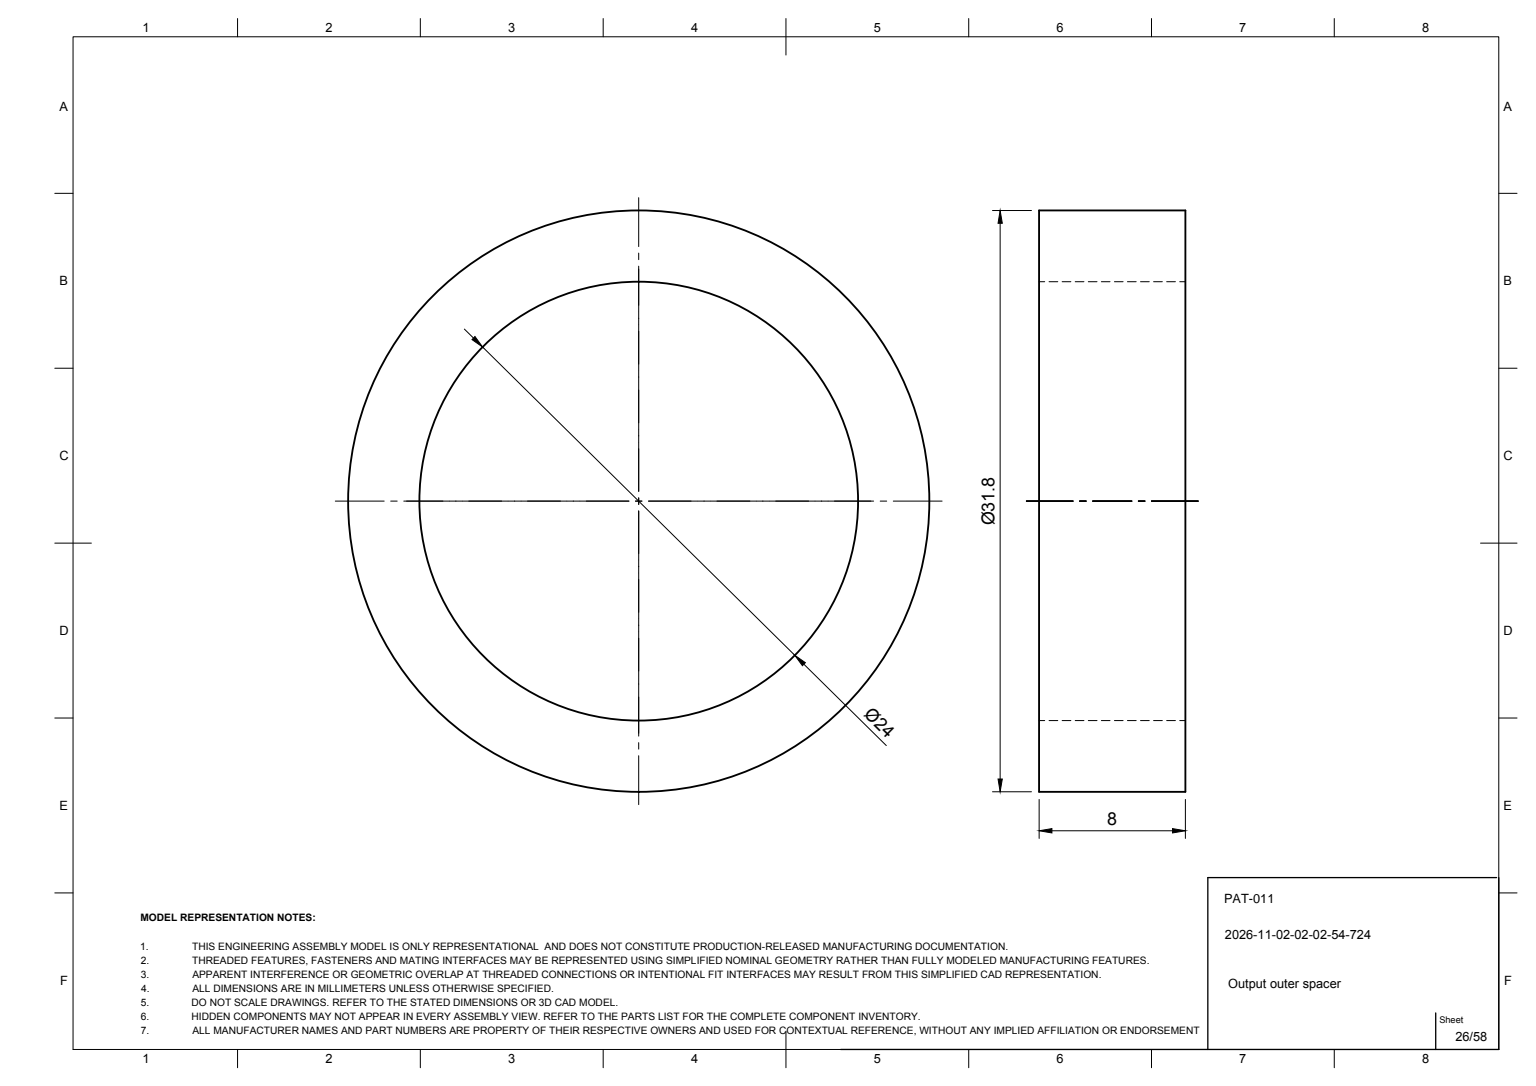
ISO-10303-21;
HEADER;
/* Generated by software containing ST-Developer
 * from STEP Tools, Inc. (www.steptools.com) 
 */

FILE_DESCRIPTION(
/* description */ ('Belt tension measurement rig'),
/* implementation_level */ '2;1');

FILE_NAME(
/* name */ 'Output outer spacer.step',
/* time_stamp */ '2026-10-28T03:24:44-07:00',
/* author */ (''),
/* organization */ (''),
/* preprocessor_version */ 'ST-DEVELOPER v20.2',
/* originating_system */ 'Autodesk Translation Framework v15.17.0.0',
/* authorisation */ '');

FILE_SCHEMA (('AUTOMOTIVE_DESIGN { 1 0 10303 214 3 1 1 }'));
ENDSEC;

DATA;
#10=MECHANICAL_DESIGN_GEOMETRIC_PRESENTATION_REPRESENTATION('',(#721),#23587);
#603=SHAPE_REPRESENTATION_RELATIONSHIP('SRR','None',#23850,#658);
#658=ADVANCED_BREP_SHAPE_REPRESENTATION('',(#791),#23548);
#721=STYLED_ITEM('',(#24225),#791);
#791=MANIFOLD_SOLID_BREP('Body1',#12226);
#954=FACE_BOUND('',#2455,.T.);
#955=FACE_BOUND('',#2457,.T.);
#1175=PLANE('',#13454);
#1176=PLANE('',#13455);
#1623=FACE_OUTER_BOUND('',#2452,.T.);
#1624=FACE_OUTER_BOUND('',#2453,.T.);
#1625=FACE_OUTER_BOUND('',#2454,.T.);
#1626=FACE_OUTER_BOUND('',#2456,.T.);
#2452=EDGE_LOOP('',(#9130,#9131,#9132,#9133));
#2453=EDGE_LOOP('',(#9134,#9135,#9136,#9137));
#2454=EDGE_LOOP('',(#9138));
#2455=EDGE_LOOP('',(#9139));
#2456=EDGE_LOOP('',(#9140));
#2457=EDGE_LOOP('',(#9141));
#3272=LINE('',#20266,#4023);
#3273=LINE('',#20272,#4024);
#4023=VECTOR('',#15969,1.2);
#4024=VECTOR('',#15976,1.59);
#4740=CIRCLE('',#13449,1.2);
#4741=CIRCLE('',#13450,1.2);
#4742=CIRCLE('',#13452,1.59);
#4743=CIRCLE('',#13453,1.59);
#5642=VERTEX_POINT('',#20263);
#5643=VERTEX_POINT('',#20265);
#5644=VERTEX_POINT('',#20269);
#5645=VERTEX_POINT('',#20271);
#6924=EDGE_CURVE('',#5642,#5642,#4740,.T.);
#6925=EDGE_CURVE('',#5642,#5643,#3272,.T.);
#6926=EDGE_CURVE('',#5643,#5643,#4741,.T.);
#6927=EDGE_CURVE('',#5644,#5644,#4742,.T.);
#6928=EDGE_CURVE('',#5644,#5645,#3273,.T.);
#6929=EDGE_CURVE('',#5645,#5645,#4743,.T.);
#9130=ORIENTED_EDGE('',*,*,#6924,.F.);
#9131=ORIENTED_EDGE('',*,*,#6925,.T.);
#9132=ORIENTED_EDGE('',*,*,#6926,.T.);
#9133=ORIENTED_EDGE('',*,*,#6925,.F.);
#9134=ORIENTED_EDGE('',*,*,#6927,.F.);
#9135=ORIENTED_EDGE('',*,*,#6928,.T.);
#9136=ORIENTED_EDGE('',*,*,#6929,.T.);
#9137=ORIENTED_EDGE('',*,*,#6928,.F.);
#9138=ORIENTED_EDGE('',*,*,#6927,.T.);
#9139=ORIENTED_EDGE('',*,*,#6924,.T.);
#9140=ORIENTED_EDGE('',*,*,#6929,.F.);
#9141=ORIENTED_EDGE('',*,*,#6926,.F.);
#11269=CYLINDRICAL_SURFACE('',#13448,1.2);
#11270=CYLINDRICAL_SURFACE('',#13451,1.59);
#11764=ADVANCED_FACE('',(#1623),#11269,.F.);
#11765=ADVANCED_FACE('',(#1624),#11270,.T.);
#11766=ADVANCED_FACE('',(#1625,#954),#1175,.T.);
#11767=ADVANCED_FACE('',(#1626,#955),#1176,.F.);
#12226=CLOSED_SHELL('',(#11764,#11765,#11766,#11767));
#13447=AXIS2_PLACEMENT_3D('',#20261,#15963,#15964);
#13448=AXIS2_PLACEMENT_3D('',#20262,#15965,#15966);
#13449=AXIS2_PLACEMENT_3D('',#20264,#15967,#15968);
#13450=AXIS2_PLACEMENT_3D('',#20267,#15970,#15971);
#13451=AXIS2_PLACEMENT_3D('',#20268,#15972,#15973);
#13452=AXIS2_PLACEMENT_3D('',#20270,#15974,#15975);
#13453=AXIS2_PLACEMENT_3D('',#20273,#15977,#15978);
#13454=AXIS2_PLACEMENT_3D('',#20274,#15979,#15980);
#13455=AXIS2_PLACEMENT_3D('',#20275,#15981,#15982);
#15963=DIRECTION('axis',(0.,0.,1.));
#15964=DIRECTION('refdir',(1.,0.,0.));
#15965=DIRECTION('center_axis',(0.,1.,0.));
#15966=DIRECTION('ref_axis',(1.,0.,0.));
#15967=DIRECTION('center_axis',(0.,-1.,0.));
#15968=DIRECTION('ref_axis',(1.,0.,0.));
#15969=DIRECTION('',(0.,-1.,0.));
#15970=DIRECTION('center_axis',(0.,-1.,0.));
#15971=DIRECTION('ref_axis',(1.,0.,0.));
#15972=DIRECTION('center_axis',(0.,1.,0.));
#15973=DIRECTION('ref_axis',(1.,0.,0.));
#15974=DIRECTION('center_axis',(0.,1.,0.));
#15975=DIRECTION('ref_axis',(1.,0.,0.));
#15976=DIRECTION('',(0.,-1.,0.));
#15977=DIRECTION('center_axis',(0.,1.,0.));
#15978=DIRECTION('ref_axis',(1.,0.,0.));
#15979=DIRECTION('center_axis',(0.,1.,0.));
#15980=DIRECTION('ref_axis',(1.,0.,0.));
#15981=DIRECTION('center_axis',(0.,1.,0.));
#15982=DIRECTION('ref_axis',(1.,0.,0.));
#20261=CARTESIAN_POINT('',(0.,0.,0.));
#20262=CARTESIAN_POINT('Origin',(10.,-0.4,7.));
#20263=CARTESIAN_POINT('',(8.8,0.4,7.));
#20264=CARTESIAN_POINT('Origin',(10.,0.4,7.));
#20265=CARTESIAN_POINT('',(8.8,-0.4,7.));
#20266=CARTESIAN_POINT('',(8.8,-0.4,7.));
#20267=CARTESIAN_POINT('Origin',(10.,-0.4,7.));
#20268=CARTESIAN_POINT('Origin',(10.,-0.4,7.));
#20269=CARTESIAN_POINT('',(8.41,0.4,7.));
#20270=CARTESIAN_POINT('Origin',(10.,0.4,7.));
#20271=CARTESIAN_POINT('',(8.41,-0.4,7.));
#20272=CARTESIAN_POINT('',(8.41,-0.4,7.));
#20273=CARTESIAN_POINT('Origin',(10.,-0.4,7.));
#20274=CARTESIAN_POINT('Origin',(10.,0.4,7.));
#20275=CARTESIAN_POINT('Origin',(10.,-0.4,7.));
#23483=UNCERTAINTY_MEASURE_WITH_UNIT(LENGTH_MEASURE(0.001),#23588,
'DISTANCE_ACCURACY_VALUE',
'Maximum model space distance between geometric entities at asserted c
onnectivities');
#23522=UNCERTAINTY_MEASURE_WITH_UNIT(LENGTH_MEASURE(0.001),#23588,
'DISTANCE_ACCURACY_VALUE',
'Maximum model space distance between geometric entities at asserted c
onnectivities');
#23548=(
GEOMETRIC_REPRESENTATION_CONTEXT(3)
GLOBAL_UNCERTAINTY_ASSIGNED_CONTEXT((#23483))
GLOBAL_UNIT_ASSIGNED_CONTEXT((#23588,#23590,#23591))
REPRESENTATION_CONTEXT('','3D')
);
#23587=(
GEOMETRIC_REPRESENTATION_CONTEXT(3)
GLOBAL_UNCERTAINTY_ASSIGNED_CONTEXT((#23522))
GLOBAL_UNIT_ASSIGNED_CONTEXT((#23588,#23590,#23591))
REPRESENTATION_CONTEXT('','3D')
);
#23588=(
LENGTH_UNIT()
NAMED_UNIT(*)
SI_UNIT(.CENTI.,.METRE.)
);
#23590=(
NAMED_UNIT(*)
PLANE_ANGLE_UNIT()
SI_UNIT($,.RADIAN.)
);
#23591=(
NAMED_UNIT(*)
SI_UNIT($,.STERADIAN.)
SOLID_ANGLE_UNIT()
);
#23617=SHAPE_DEFINITION_REPRESENTATION(#23686,#23850);
#23686=PRODUCT_DEFINITION_SHAPE('',$,#23915);
#23850=SHAPE_REPRESENTATION('',(#13447),#23548);
#23889=PRODUCT_DEFINITION_CONTEXT('part definition',#24083,'design');
#23915=PRODUCT_DEFINITION('Output outer spacer','Output outer spacer',#23979,
#23889);
#23979=PRODUCT_DEFINITION_FORMATION('',$,#24110);
#24083=APPLICATION_CONTEXT(
'Core Data for Automotive Mechanical Design Process');
#24084=PRODUCT_CONTEXT('part definition',#24083,'mechanical');
#24110=PRODUCT('Output outer spacer','Output outer spacer',
'Output outer spacer',(#24084));
#24219=COLOUR_RGB('Off White',0.89,0.88,0.83);
#24220=FILL_AREA_STYLE_COLOUR('',#24219);
#24221=FILL_AREA_STYLE('',(#24220));
#24222=SURFACE_STYLE_FILL_AREA(#24221);
#24223=SURFACE_SIDE_STYLE('',(#24222));
#24224=SURFACE_STYLE_USAGE(.BOTH.,#24223);
#24225=PRESENTATION_STYLE_ASSIGNMENT((#24224));
ENDSEC;
END-ISO-10303-21;
